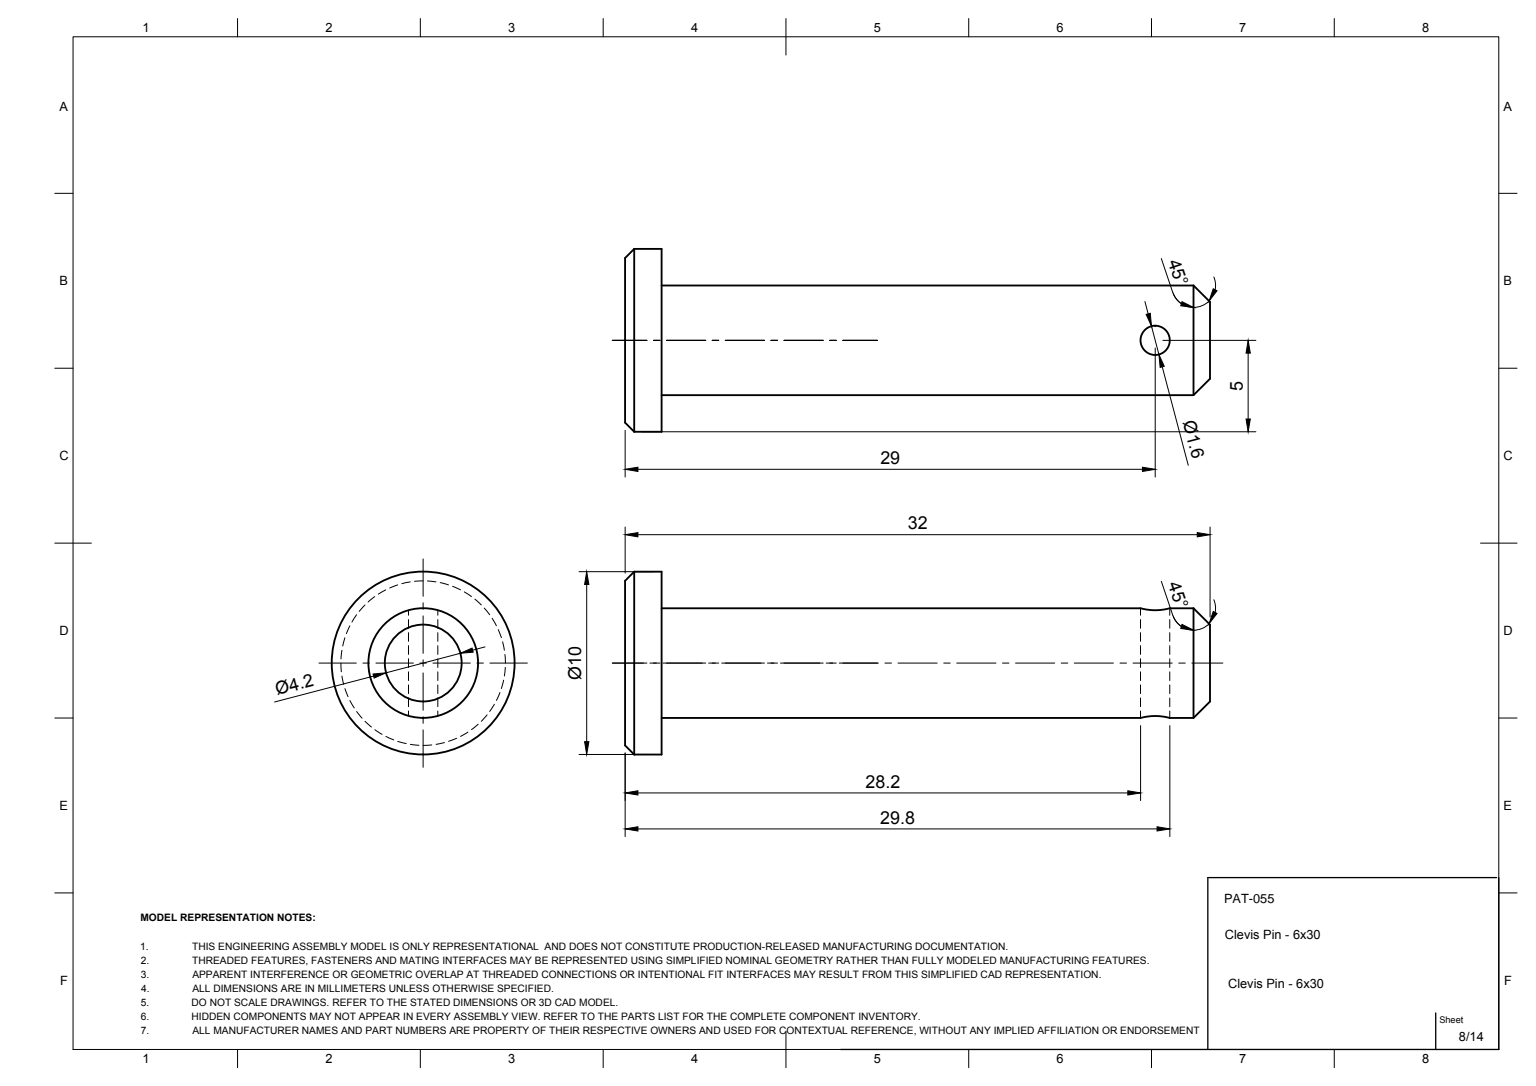
ISO-10303-21;
HEADER;
/* Generated by software containing ST-Developer
 * from STEP Tools, Inc. (www.steptools.com) 
 */

FILE_DESCRIPTION(
/* description */ ('Hinged panel with latch'),
/* implementation_level */ '2;1');

FILE_NAME(
/* name */ 'Clevis Pin - 6x30.step',
/* time_stamp */ '2026-10-27T20:36:01-07:00',
/* author */ (''),
/* organization */ (''),
/* preprocessor_version */ 'ST-DEVELOPER v20.2',
/* originating_system */ 'Autodesk Translation Framework v15.17.0.0',
/* authorisation */ '');

FILE_SCHEMA (('AUTOMOTIVE_DESIGN { 1 0 10303 214 3 1 1 }'));
ENDSEC;

DATA;
#10=MECHANICAL_DESIGN_GEOMETRIC_PRESENTATION_REPRESENTATION('',(#299),#6743);
#240=CONICAL_SURFACE('',#4092,0.475,0.785398163397448);
#241=CONICAL_SURFACE('',#4100,0.255,0.785398163397449);
#258=B_SPLINE_CURVE_WITH_KNOTS('',3,(#5867,#5868,#5869,#5870,#5871,#5872,
#5873,#5874,#5875,#5876),.UNSPECIFIED.,.F.,.F.,(4,2,2,2,4),(0.,0.0302963256060356,
0.0605926512120712,0.090883446720838,0.121174242229605),.UNSPECIFIED.);
#259=B_SPLINE_CURVE_WITH_KNOTS('',3,(#5879,#5880,#5881,#5882,#5883,#5884,
#5885,#5886,#5887,#5888,#5889,#5890,#5891,#5892,#5893,#5894,#5895,#5896,
#5897,#5898,#5899,#5900,#5901,#5902,#5903,#5904,#5905,#5906,#5907,#5908,
#5909,#5910,#5911,#5912),.UNSPECIFIED.,.T.,.F.,(4,2,2,2,2,2,2,2,2,2,2,2,
2,2,2,2,4),(0.,0.0302963256060358,0.0605926512120716,0.0908834467208383,
0.121174242229605,0.151465037738372,0.181755833247138,0.212052158853174,
0.24234848445921,0.272644810065246,0.302941135671282,0.333231931180048,
0.363522726688815,0.393813522197582,0.424104317706349,0.454400643312384,
0.48469696891842),.UNSPECIFIED.);
#260=B_SPLINE_CURVE_WITH_KNOTS('',3,(#5914,#5915,#5916,#5917,#5918,#5919,
#5920,#5921,#5922,#5923),.UNSPECIFIED.,.F.,.F.,(4,2,2,2,4),(0.363522726688815,
0.393813522197581,0.424104317706348,0.454400643312384,0.48469696891842),
 .UNSPECIFIED.);
#261=B_SPLINE_CURVE_WITH_KNOTS('',3,(#5924,#5925,#5926,#5927,#5928,#5929,
#5930,#5931,#5932,#5933,#5934,#5935,#5936,#5937,#5938,#5939,#5940,#5941),
 .UNSPECIFIED.,.F.,.F.,(4,2,2,2,2,2,2,2,4),(0.121174242229605,0.151465037738371,
0.181755833247138,0.212052158853174,0.24234848445921,0.272644810065246,
0.302941135671281,0.333231931180048,0.363522726688815),.UNSPECIFIED.);
#267=SHAPE_REPRESENTATION_RELATIONSHIP('SRR','None',#6842,#283);
#283=ADVANCED_BREP_SHAPE_REPRESENTATION('',(#315),#6728);
#299=STYLED_ITEM('',(#7003),#315);
#315=MANIFOLD_SOLID_BREP('Body1',#3801);
#339=FACE_BOUND('',#819,.T.);
#340=FACE_BOUND('',#821,.T.);
#434=PLANE('',#4090);
#435=PLANE('',#4096);
#436=PLANE('',#4102);
#594=FACE_OUTER_BOUND('',#814,.T.);
#595=FACE_OUTER_BOUND('',#815,.T.);
#596=FACE_OUTER_BOUND('',#816,.T.);
#597=FACE_OUTER_BOUND('',#817,.T.);
#598=FACE_OUTER_BOUND('',#818,.T.);
#599=FACE_OUTER_BOUND('',#820,.T.);
#600=FACE_OUTER_BOUND('',#822,.T.);
#601=FACE_OUTER_BOUND('',#823,.T.);
#814=EDGE_LOOP('',(#2980,#2981,#2982,#2983,#2984,#2985));
#815=EDGE_LOOP('',(#2986));
#816=EDGE_LOOP('',(#2987,#2988,#2989,#2990));
#817=EDGE_LOOP('',(#2991,#2992,#2993,#2994));
#818=EDGE_LOOP('',(#2995));
#819=EDGE_LOOP('',(#2996));
#820=EDGE_LOOP('',(#2997,#2998,#2999,#3000,#3001,#3002,#3003,#3004,#3005));
#821=EDGE_LOOP('',(#3006));
#822=EDGE_LOOP('',(#3007,#3008,#3009,#3010));
#823=EDGE_LOOP('',(#3011));
#1159=LINE('',#5878,#1517);
#1160=LINE('',#5948,#1518);
#1161=LINE('',#5952,#1519);
#1162=LINE('',#5959,#1520);
#1163=LINE('',#5960,#1521);
#1164=LINE('',#5964,#1522);
#1517=VECTOR('',#4733,0.08);
#1518=VECTOR('',#4742,0.475);
#1519=VECTOR('',#4747,0.5);
#1520=VECTOR('',#4756,0.3);
#1521=VECTOR('',#4757,0.3);
#1522=VECTOR('',#4762,0.255);
#1716=CIRCLE('',#4091,0.45);
#1717=CIRCLE('',#4093,0.5);
#1718=CIRCLE('',#4095,0.5);
#1719=CIRCLE('',#4097,0.3);
#1720=CIRCLE('',#4099,0.3);
#1721=CIRCLE('',#4101,0.21);
#1921=VERTEX_POINT('',#5865);
#1922=VERTEX_POINT('',#5866);
#1923=VERTEX_POINT('',#5877);
#1924=VERTEX_POINT('',#5913);
#1925=VERTEX_POINT('',#5943);
#1926=VERTEX_POINT('',#5946);
#1927=VERTEX_POINT('',#5950);
#1928=VERTEX_POINT('',#5954);
#1929=VERTEX_POINT('',#5957);
#1930=VERTEX_POINT('',#5962);
#2302=EDGE_CURVE('',#1921,#1922,#258,.T.);
#2303=EDGE_CURVE('',#1921,#1923,#1159,.T.);
#2304=EDGE_CURVE('',#1923,#1923,#259,.T.);
#2305=EDGE_CURVE('',#1924,#1921,#260,.T.);
#2306=EDGE_CURVE('',#1922,#1924,#261,.T.);
#2307=EDGE_CURVE('',#1925,#1925,#1716,.T.);
#2308=EDGE_CURVE('',#1926,#1926,#1717,.T.);
#2309=EDGE_CURVE('',#1926,#1925,#1160,.T.);
#2310=EDGE_CURVE('',#1927,#1927,#1718,.T.);
#2311=EDGE_CURVE('',#1927,#1926,#1161,.T.);
#2312=EDGE_CURVE('',#1928,#1928,#1719,.T.);
#2313=EDGE_CURVE('',#1929,#1929,#1720,.T.);
#2314=EDGE_CURVE('',#1929,#1922,#1162,.T.);
#2315=EDGE_CURVE('',#1924,#1928,#1163,.T.);
#2316=EDGE_CURVE('',#1930,#1930,#1721,.T.);
#2317=EDGE_CURVE('',#1930,#1929,#1164,.T.);
#2980=ORIENTED_EDGE('',*,*,#2302,.F.);
#2981=ORIENTED_EDGE('',*,*,#2303,.T.);
#2982=ORIENTED_EDGE('',*,*,#2304,.F.);
#2983=ORIENTED_EDGE('',*,*,#2303,.F.);
#2984=ORIENTED_EDGE('',*,*,#2305,.F.);
#2985=ORIENTED_EDGE('',*,*,#2306,.F.);
#2986=ORIENTED_EDGE('',*,*,#2307,.F.);
#2987=ORIENTED_EDGE('',*,*,#2308,.F.);
#2988=ORIENTED_EDGE('',*,*,#2309,.T.);
#2989=ORIENTED_EDGE('',*,*,#2307,.T.);
#2990=ORIENTED_EDGE('',*,*,#2309,.F.);
#2991=ORIENTED_EDGE('',*,*,#2310,.F.);
#2992=ORIENTED_EDGE('',*,*,#2311,.T.);
#2993=ORIENTED_EDGE('',*,*,#2308,.T.);
#2994=ORIENTED_EDGE('',*,*,#2311,.F.);
#2995=ORIENTED_EDGE('',*,*,#2310,.T.);
#2996=ORIENTED_EDGE('',*,*,#2312,.F.);
#2997=ORIENTED_EDGE('',*,*,#2313,.F.);
#2998=ORIENTED_EDGE('',*,*,#2314,.T.);
#2999=ORIENTED_EDGE('',*,*,#2306,.T.);
#3000=ORIENTED_EDGE('',*,*,#2315,.T.);
#3001=ORIENTED_EDGE('',*,*,#2312,.T.);
#3002=ORIENTED_EDGE('',*,*,#2315,.F.);
#3003=ORIENTED_EDGE('',*,*,#2305,.T.);
#3004=ORIENTED_EDGE('',*,*,#2302,.T.);
#3005=ORIENTED_EDGE('',*,*,#2314,.F.);
#3006=ORIENTED_EDGE('',*,*,#2304,.T.);
#3007=ORIENTED_EDGE('',*,*,#2316,.F.);
#3008=ORIENTED_EDGE('',*,*,#2317,.T.);
#3009=ORIENTED_EDGE('',*,*,#2313,.T.);
#3010=ORIENTED_EDGE('',*,*,#2317,.F.);
#3011=ORIENTED_EDGE('',*,*,#2316,.T.);
#3565=CYLINDRICAL_SURFACE('',#4089,0.08);
#3566=CYLINDRICAL_SURFACE('',#4094,0.5);
#3567=CYLINDRICAL_SURFACE('',#4098,0.3);
#3663=ADVANCED_FACE('',(#594),#3565,.F.);
#3664=ADVANCED_FACE('',(#595),#434,.T.);
#3665=ADVANCED_FACE('',(#596),#240,.T.);
#3666=ADVANCED_FACE('',(#597),#3566,.T.);
#3667=ADVANCED_FACE('',(#598,#339),#435,.T.);
#3668=ADVANCED_FACE('',(#599,#340),#3567,.T.);
#3669=ADVANCED_FACE('',(#600),#241,.T.);
#3670=ADVANCED_FACE('',(#601),#436,.T.);
#3801=CLOSED_SHELL('',(#3663,#3664,#3665,#3666,#3667,#3668,#3669,#3670));
#4088=AXIS2_PLACEMENT_3D('',#5863,#4729,#4730);
#4089=AXIS2_PLACEMENT_3D('',#5864,#4731,#4732);
#4090=AXIS2_PLACEMENT_3D('',#5942,#4734,#4735);
#4091=AXIS2_PLACEMENT_3D('',#5944,#4736,#4737);
#4092=AXIS2_PLACEMENT_3D('',#5945,#4738,#4739);
#4093=AXIS2_PLACEMENT_3D('',#5947,#4740,#4741);
#4094=AXIS2_PLACEMENT_3D('',#5949,#4743,#4744);
#4095=AXIS2_PLACEMENT_3D('',#5951,#4745,#4746);
#4096=AXIS2_PLACEMENT_3D('',#5953,#4748,#4749);
#4097=AXIS2_PLACEMENT_3D('',#5955,#4750,#4751);
#4098=AXIS2_PLACEMENT_3D('',#5956,#4752,#4753);
#4099=AXIS2_PLACEMENT_3D('',#5958,#4754,#4755);
#4100=AXIS2_PLACEMENT_3D('',#5961,#4758,#4759);
#4101=AXIS2_PLACEMENT_3D('',#5963,#4760,#4761);
#4102=AXIS2_PLACEMENT_3D('',#5965,#4763,#4764);
#4729=DIRECTION('axis',(0.,0.,1.));
#4730=DIRECTION('refdir',(1.,0.,0.));
#4731=DIRECTION('center_axis',(1.,0.,0.));
#4732=DIRECTION('ref_axis',(0.,0.,-1.));
#4733=DIRECTION('',(1.,0.,0.));
#4734=DIRECTION('center_axis',(0.,1.,0.));
#4735=DIRECTION('ref_axis',(0.,0.,1.));
#4736=DIRECTION('center_axis',(0.,-1.,0.));
#4737=DIRECTION('ref_axis',(1.,0.,0.));
#4738=DIRECTION('center_axis',(0.,-1.,0.));
#4739=DIRECTION('ref_axis',(1.,0.,0.));
#4740=DIRECTION('center_axis',(0.,-1.,0.));
#4741=DIRECTION('ref_axis',(1.,0.,0.));
#4742=DIRECTION('',(0.707106781186547,0.707106781186548,8.65956056235493E-17));
#4743=DIRECTION('center_axis',(0.,-1.,0.));
#4744=DIRECTION('ref_axis',(1.,0.,0.));
#4745=DIRECTION('center_axis',(0.,-1.,0.));
#4746=DIRECTION('ref_axis',(1.,0.,0.));
#4747=DIRECTION('',(0.,1.,0.));
#4748=DIRECTION('center_axis',(0.,-1.,0.));
#4749=DIRECTION('ref_axis',(0.,0.,-1.));
#4750=DIRECTION('center_axis',(0.,-1.,0.));
#4751=DIRECTION('ref_axis',(1.,0.,0.));
#4752=DIRECTION('center_axis',(0.,-1.,0.));
#4753=DIRECTION('ref_axis',(1.,0.,0.));
#4754=DIRECTION('center_axis',(0.,-1.,0.));
#4755=DIRECTION('ref_axis',(1.,0.,0.));
#4756=DIRECTION('',(0.,1.,0.));
#4757=DIRECTION('',(0.,1.,0.));
#4758=DIRECTION('center_axis',(0.,1.,0.));
#4759=DIRECTION('ref_axis',(1.,0.,0.));
#4760=DIRECTION('center_axis',(0.,-1.,0.));
#4761=DIRECTION('ref_axis',(1.,0.,0.));
#4762=DIRECTION('',(-0.707106781186548,0.707106781186547,-8.65956056235494E-17));
#4763=DIRECTION('center_axis',(0.,-1.,0.));
#4764=DIRECTION('ref_axis',(0.,0.,-1.));
#5863=CARTESIAN_POINT('',(0.,0.,0.));
#5864=CARTESIAN_POINT('Origin',(0.,-2.7,0.));
#5865=CARTESIAN_POINT('',(-0.289136645896019,-2.7,0.08));
#5866=CARTESIAN_POINT('',(-0.3,-2.78,-2.27065106771523E-17));
#5867=CARTESIAN_POINT('Ctrl Pts',(-0.289136645896019,-2.7,0.08));
#5868=CARTESIAN_POINT('Ctrl Pts',(-0.289136645896019,-2.71009877520201,
0.08));
#5869=CARTESIAN_POINT('Ctrl Pts',(-0.289720927595908,-2.72083518625944,
0.0779717130936404));
#5870=CARTESIAN_POINT('Ctrl Pts',(-0.291799203044223,-2.74052980652726,
0.0697927537456149));
#5871=CARTESIAN_POINT('Ctrl Pts',(-0.293259762986909,-2.74949254880105,
0.0636445361887959));
#5872=CARTESIAN_POINT('Ctrl Pts',(-0.295976783522942,-2.76364324458222,
0.0494938404076284));
#5873=CARTESIAN_POINT('Ctrl Pts',(-0.297414335384467,-2.76979246713824,
0.0405305642602551));
#5874=CARTESIAN_POINT('Ctrl Pts',(-0.299439403644655,-2.77797216257078,
0.0208340363410407));
#5875=CARTESIAN_POINT('Ctrl Pts',(-0.3,-2.78,0.0100969318362556));
#5876=CARTESIAN_POINT('Ctrl Pts',(-0.3,-2.78,5.20417042793042E-18));
#5877=CARTESIAN_POINT('',(0.289136645896019,-2.7,0.08));
#5878=CARTESIAN_POINT('',(0.,-2.7,0.08));
#5879=CARTESIAN_POINT('Ctrl Pts',(0.289136645896019,-2.7,0.08));
#5880=CARTESIAN_POINT('Ctrl Pts',(0.289136645896019,-2.68990122479799,0.08));
#5881=CARTESIAN_POINT('Ctrl Pts',(0.289720927595908,-2.67916481374056,0.0779717130936404));
#5882=CARTESIAN_POINT('Ctrl Pts',(0.291799203044223,-2.65947019347274,0.0697927537456147));
#5883=CARTESIAN_POINT('Ctrl Pts',(0.293259762986909,-2.65050745119895,0.0636445361887959));
#5884=CARTESIAN_POINT('Ctrl Pts',(0.295976783522942,-2.63635675541778,0.0494938404076283));
#5885=CARTESIAN_POINT('Ctrl Pts',(0.297414335384467,-2.63020753286176,0.0405305642602551));
#5886=CARTESIAN_POINT('Ctrl Pts',(0.299439403644655,-2.62202783742922,0.0208340363410406));
#5887=CARTESIAN_POINT('Ctrl Pts',(0.3,-2.62,0.0100969318362555));
#5888=CARTESIAN_POINT('Ctrl Pts',(0.3,-2.62,-0.0100969318362556));
#5889=CARTESIAN_POINT('Ctrl Pts',(0.299439403644655,-2.62202783742922,-0.0208340363410406));
#5890=CARTESIAN_POINT('Ctrl Pts',(0.297414335384467,-2.63020753286176,-0.0405305642602551));
#5891=CARTESIAN_POINT('Ctrl Pts',(0.295976783522942,-2.63635675541778,-0.0494938404076283));
#5892=CARTESIAN_POINT('Ctrl Pts',(0.293259762986909,-2.65050745119895,-0.0636445361887959));
#5893=CARTESIAN_POINT('Ctrl Pts',(0.291799203044223,-2.65947019347274,-0.0697927537456147));
#5894=CARTESIAN_POINT('Ctrl Pts',(0.289720927595908,-2.67916481374056,-0.0779717130936403));
#5895=CARTESIAN_POINT('Ctrl Pts',(0.289136645896019,-2.68990122479799,-0.08));
#5896=CARTESIAN_POINT('Ctrl Pts',(0.289136645896019,-2.71009877520201,-0.08));
#5897=CARTESIAN_POINT('Ctrl Pts',(0.289720927595908,-2.72083518625944,-0.0779717130936404));
#5898=CARTESIAN_POINT('Ctrl Pts',(0.291799203044223,-2.74052980652726,-0.0697927537456147));
#5899=CARTESIAN_POINT('Ctrl Pts',(0.293259762986909,-2.74949254880105,-0.0636445361887959));
#5900=CARTESIAN_POINT('Ctrl Pts',(0.295976783522942,-2.76364324458222,-0.0494938404076283));
#5901=CARTESIAN_POINT('Ctrl Pts',(0.297414335384467,-2.76979246713824,-0.0405305642602551));
#5902=CARTESIAN_POINT('Ctrl Pts',(0.299439403644655,-2.77797216257078,-0.0208340363410406));
#5903=CARTESIAN_POINT('Ctrl Pts',(0.3,-2.78,-0.0100969318362555));
#5904=CARTESIAN_POINT('Ctrl Pts',(0.3,-2.78,0.0100969318362556));
#5905=CARTESIAN_POINT('Ctrl Pts',(0.299439403644655,-2.77797216257078,0.0208340363410407));
#5906=CARTESIAN_POINT('Ctrl Pts',(0.297414335384467,-2.76979246713824,0.0405305642602551));
#5907=CARTESIAN_POINT('Ctrl Pts',(0.295976783522942,-2.76364324458222,0.0494938404076284));
#5908=CARTESIAN_POINT('Ctrl Pts',(0.293259762986909,-2.74949254880105,0.0636445361887959));
#5909=CARTESIAN_POINT('Ctrl Pts',(0.291799203044223,-2.74052980652726,0.0697927537456149));
#5910=CARTESIAN_POINT('Ctrl Pts',(0.289720927595908,-2.72083518625944,0.0779717130936404));
#5911=CARTESIAN_POINT('Ctrl Pts',(0.289136645896019,-2.71009877520201,0.08));
#5912=CARTESIAN_POINT('Ctrl Pts',(0.289136645896019,-2.7,0.08));
#5913=CARTESIAN_POINT('',(-0.3,-2.62,-3.65842984849668E-17));
#5914=CARTESIAN_POINT('Ctrl Pts',(-0.3,-2.62,-3.81639164714898E-17));
#5915=CARTESIAN_POINT('Ctrl Pts',(-0.3,-2.62,0.0100969318362555));
#5916=CARTESIAN_POINT('Ctrl Pts',(-0.299439403644655,-2.62202783742922,
0.0208340363410406));
#5917=CARTESIAN_POINT('Ctrl Pts',(-0.297414335384467,-2.63020753286176,
0.040530564260255));
#5918=CARTESIAN_POINT('Ctrl Pts',(-0.295976783522942,-2.63635675541778,
0.0494938404076283));
#5919=CARTESIAN_POINT('Ctrl Pts',(-0.293259762986909,-2.65050745119895,
0.0636445361887959));
#5920=CARTESIAN_POINT('Ctrl Pts',(-0.291799203044223,-2.65947019347274,
0.0697927537456147));
#5921=CARTESIAN_POINT('Ctrl Pts',(-0.289720927595908,-2.67916481374056,
0.0779717130936404));
#5922=CARTESIAN_POINT('Ctrl Pts',(-0.289136645896019,-2.68990122479799,
0.08));
#5923=CARTESIAN_POINT('Ctrl Pts',(-0.289136645896019,-2.7,0.08));
#5924=CARTESIAN_POINT('Ctrl Pts',(-0.3,-2.78,-6.93889390390723E-18));
#5925=CARTESIAN_POINT('Ctrl Pts',(-0.3,-2.78,-0.0100969318362556));
#5926=CARTESIAN_POINT('Ctrl Pts',(-0.299439403644655,-2.77797216257078,
-0.0208340363410406));
#5927=CARTESIAN_POINT('Ctrl Pts',(-0.297414335384467,-2.76979246713824,
-0.0405305642602551));
#5928=CARTESIAN_POINT('Ctrl Pts',(-0.295976783522942,-2.76364324458222,
-0.0494938404076283));
#5929=CARTESIAN_POINT('Ctrl Pts',(-0.293259762986909,-2.74949254880105,
-0.0636445361887959));
#5930=CARTESIAN_POINT('Ctrl Pts',(-0.291799203044223,-2.74052980652726,
-0.0697927537456147));
#5931=CARTESIAN_POINT('Ctrl Pts',(-0.289720927595908,-2.72083518625944,
-0.0779717130936403));
#5932=CARTESIAN_POINT('Ctrl Pts',(-0.289136645896019,-2.71009877520201,
-0.08));
#5933=CARTESIAN_POINT('Ctrl Pts',(-0.289136645896019,-2.68990122479799,
-0.08));
#5934=CARTESIAN_POINT('Ctrl Pts',(-0.289720927595908,-2.67916481374056,
-0.0779717130936403));
#5935=CARTESIAN_POINT('Ctrl Pts',(-0.291799203044223,-2.65947019347274,
-0.0697927537456147));
#5936=CARTESIAN_POINT('Ctrl Pts',(-0.293259762986909,-2.65050745119895,
-0.0636445361887959));
#5937=CARTESIAN_POINT('Ctrl Pts',(-0.295976783522942,-2.63635675541778,
-0.0494938404076283));
#5938=CARTESIAN_POINT('Ctrl Pts',(-0.297414335384467,-2.63020753286176,
-0.0405305642602551));
#5939=CARTESIAN_POINT('Ctrl Pts',(-0.299439403644655,-2.62202783742922,
-0.0208340363410406));
#5940=CARTESIAN_POINT('Ctrl Pts',(-0.3,-2.62,-0.0100969318362556));
#5941=CARTESIAN_POINT('Ctrl Pts',(-0.3,-2.62,-1.56125112837913E-17));
#5942=CARTESIAN_POINT('Origin',(0.45,0.2,0.));
#5943=CARTESIAN_POINT('',(-0.45,0.2,-5.51091059616309E-17));
#5944=CARTESIAN_POINT('Origin',(0.,0.2,0.));
#5945=CARTESIAN_POINT('Origin',(0.,0.175,0.));
#5946=CARTESIAN_POINT('',(-0.5,0.15,-6.12323399573676E-17));
#5947=CARTESIAN_POINT('Origin',(0.,0.15,0.));
#5948=CARTESIAN_POINT('',(-0.475,0.175,-5.81707229594993E-17));
#5949=CARTESIAN_POINT('Origin',(0.,0.0750000000000002,0.));
#5950=CARTESIAN_POINT('',(-0.5,0.,-6.12323399573677E-17));
#5951=CARTESIAN_POINT('Origin',(0.,0.,0.));
#5952=CARTESIAN_POINT('',(-0.5,0.0750000000000002,-6.12323399573677E-17));
#5953=CARTESIAN_POINT('Origin',(0.3,0.,0.));
#5954=CARTESIAN_POINT('',(-0.3,0.,-3.67394039744206E-17));
#5955=CARTESIAN_POINT('Origin',(0.,0.,0.));
#5956=CARTESIAN_POINT('Origin',(0.,-1.455,0.));
#5957=CARTESIAN_POINT('',(-0.3,-2.91,-3.67394039744206E-17));
#5958=CARTESIAN_POINT('Origin',(0.,-2.91,0.));
#5959=CARTESIAN_POINT('',(-0.3,-1.455,-3.67394039744206E-17));
#5960=CARTESIAN_POINT('',(-0.3,-1.455,-3.67394039744206E-17));
#5961=CARTESIAN_POINT('Origin',(0.,-2.955,0.));
#5962=CARTESIAN_POINT('',(-0.21,-3.,-2.57175827820944E-17));
#5963=CARTESIAN_POINT('Origin',(0.,-3.,0.));
#5964=CARTESIAN_POINT('',(-0.255,-2.955,-3.12284933782575E-17));
#5965=CARTESIAN_POINT('Origin',(0.,-3.,0.));
#6707=UNCERTAINTY_MEASURE_WITH_UNIT(LENGTH_MEASURE(0.001),#6744,
'DISTANCE_ACCURACY_VALUE',
'Maximum model space distance between geometric entities at asserted c
onnectivities');
#6722=UNCERTAINTY_MEASURE_WITH_UNIT(LENGTH_MEASURE(0.001),#6744,
'DISTANCE_ACCURACY_VALUE',
'Maximum model space distance between geometric entities at asserted c
onnectivities');
#6728=(
GEOMETRIC_REPRESENTATION_CONTEXT(3)
GLOBAL_UNCERTAINTY_ASSIGNED_CONTEXT((#6707))
GLOBAL_UNIT_ASSIGNED_CONTEXT((#6744,#6746,#6747))
REPRESENTATION_CONTEXT('','3D')
);
#6743=(
GEOMETRIC_REPRESENTATION_CONTEXT(3)
GLOBAL_UNCERTAINTY_ASSIGNED_CONTEXT((#6722))
GLOBAL_UNIT_ASSIGNED_CONTEXT((#6744,#6746,#6747))
REPRESENTATION_CONTEXT('','3D')
);
#6744=(
LENGTH_UNIT()
NAMED_UNIT(*)
SI_UNIT(.CENTI.,.METRE.)
);
#6746=(
NAMED_UNIT(*)
PLANE_ANGLE_UNIT()
SI_UNIT($,.RADIAN.)
);
#6747=(
NAMED_UNIT(*)
SI_UNIT($,.STERADIAN.)
SOLID_ANGLE_UNIT()
);
#6753=SHAPE_DEFINITION_REPRESENTATION(#6773,#6842);
#6773=PRODUCT_DEFINITION_SHAPE('',$,#6863);
#6842=SHAPE_REPRESENTATION('',(#4088),#6728);
#6857=PRODUCT_DEFINITION_CONTEXT('part definition',#6919,'design');
#6863=PRODUCT_DEFINITION('Clevis Pin - 6x30','Clevis Pin - 6x30',#6883,
#6857);
#6883=PRODUCT_DEFINITION_FORMATION('',$,#6926);
#6919=APPLICATION_CONTEXT(
'Core Data for Automotive Mechanical Design Process');
#6920=PRODUCT_CONTEXT('part definition',#6919,'mechanical');
#6926=PRODUCT('Clevis Pin - 6x30','Clevis Pin - 6x30',
'Clevis Pin - 6x30',(#6920));
#6997=COLOUR_RGB('Grey',0.48,0.52,0.57);
#6998=FILL_AREA_STYLE_COLOUR('',#6997);
#6999=FILL_AREA_STYLE('',(#6998));
#7000=SURFACE_STYLE_FILL_AREA(#6999);
#7001=SURFACE_SIDE_STYLE('',(#7000));
#7002=SURFACE_STYLE_USAGE(.BOTH.,#7001);
#7003=PRESENTATION_STYLE_ASSIGNMENT((#7002));
ENDSEC;
END-ISO-10303-21;
